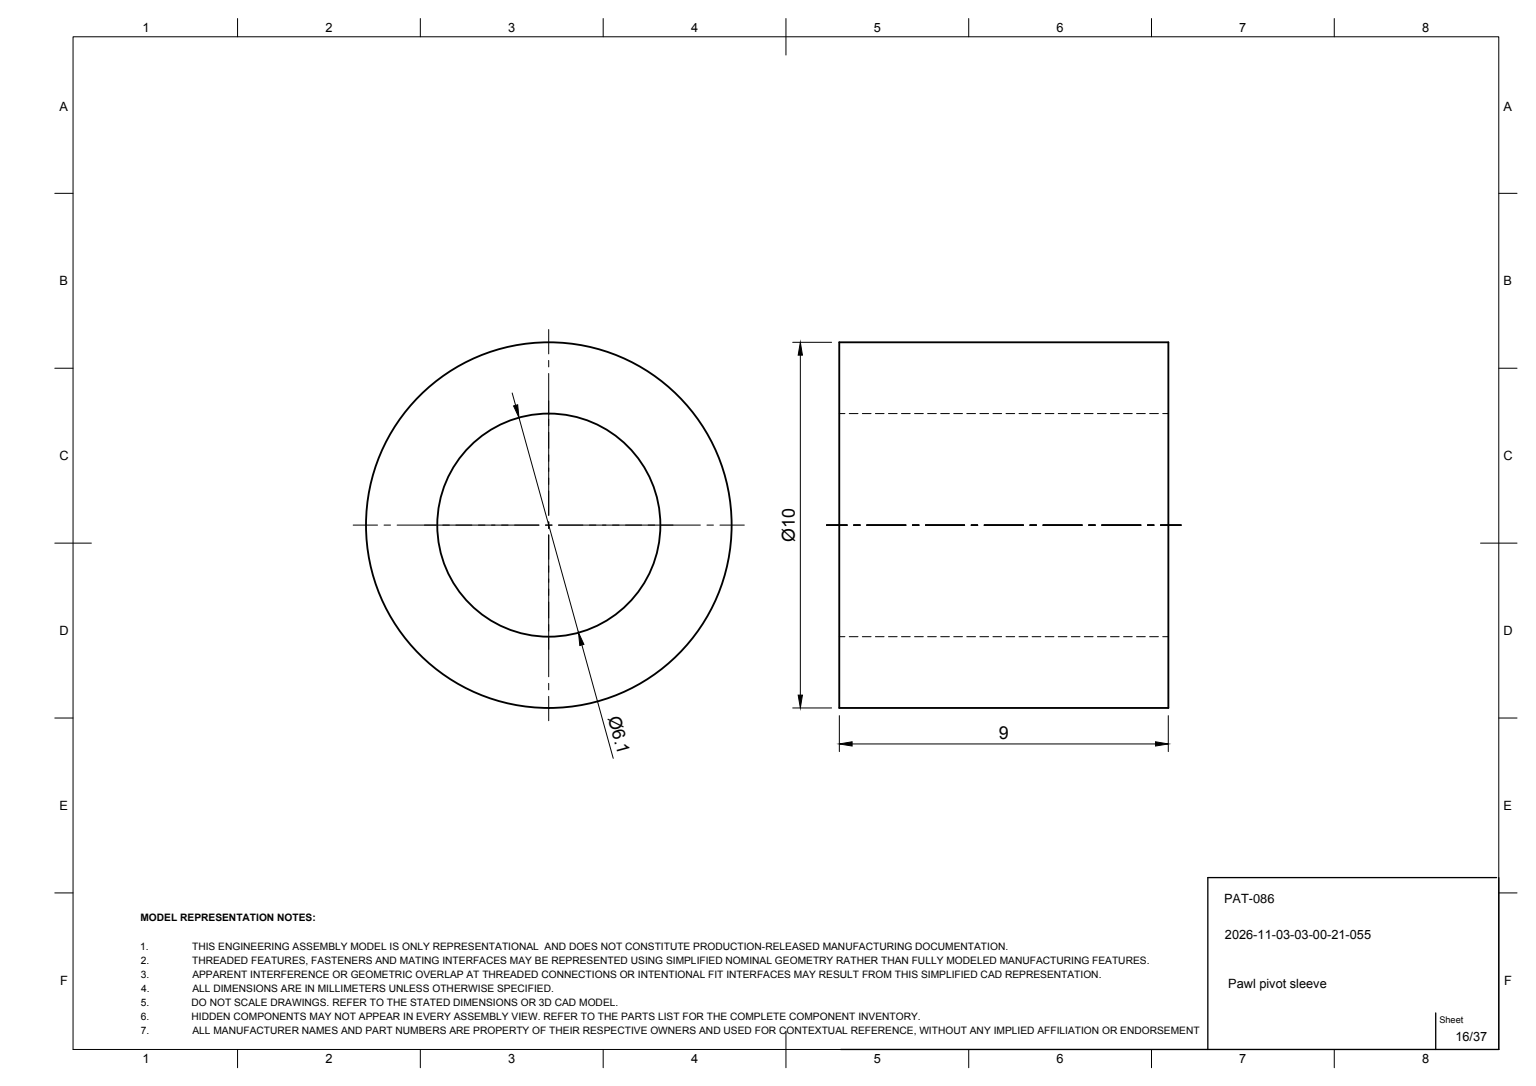
ISO-10303-21;
HEADER;
/* Generated by software containing ST-Developer
 * from STEP Tools, Inc. (www.steptools.com) 
 */

FILE_DESCRIPTION(
/* description */ ('Ratchet and pawl hand winch drum'),
/* implementation_level */ '2;1');

FILE_NAME(
/* name */ 'Pawl pivot sleeve.step',
/* time_stamp */ '2026-10-27T12:42:58-07:00',
/* author */ (''),
/* organization */ (''),
/* preprocessor_version */ 'ST-DEVELOPER v20.2',
/* originating_system */ 'Autodesk Translation Framework v15.17.0.0',
/* authorisation */ '');

FILE_SCHEMA (('AUTOMOTIVE_DESIGN { 1 0 10303 214 3 1 1 }'));
ENDSEC;

DATA;
#10=MECHANICAL_DESIGN_GEOMETRIC_PRESENTATION_REPRESENTATION('',(#400),#11801);
#332=SHAPE_REPRESENTATION_RELATIONSHIP('SRR','None',#11958,#366);
#366=ADVANCED_BREP_SHAPE_REPRESENTATION('',(#435),#11775);
#400=STYLED_ITEM('',(#12227),#435);
#435=MANIFOLD_SOLID_BREP('Body1',#6277);
#525=FACE_BOUND('',#1373,.T.);
#526=FACE_BOUND('',#1375,.T.);
#662=PLANE('',#6892);
#663=PLANE('',#6893);
#945=FACE_OUTER_BOUND('',#1370,.T.);
#946=FACE_OUTER_BOUND('',#1371,.T.);
#947=FACE_OUTER_BOUND('',#1372,.T.);
#948=FACE_OUTER_BOUND('',#1374,.T.);
#1370=EDGE_LOOP('',(#4679,#4680,#4681,#4682));
#1371=EDGE_LOOP('',(#4683,#4684,#4685,#4686));
#1372=EDGE_LOOP('',(#4687));
#1373=EDGE_LOOP('',(#4688));
#1374=EDGE_LOOP('',(#4689));
#1375=EDGE_LOOP('',(#4690));
#1825=LINE('',#9710,#2336);
#1826=LINE('',#9716,#2337);
#2336=VECTOR('',#7904,0.305);
#2337=VECTOR('',#7911,0.5);
#2807=CIRCLE('',#6887,0.305);
#2808=CIRCLE('',#6888,0.305);
#2809=CIRCLE('',#6890,0.5);
#2810=CIRCLE('',#6891,0.5);
#3086=VERTEX_POINT('',#9707);
#3087=VERTEX_POINT('',#9709);
#3088=VERTEX_POINT('',#9713);
#3089=VERTEX_POINT('',#9715);
#3683=EDGE_CURVE('',#3086,#3086,#2807,.T.);
#3684=EDGE_CURVE('',#3086,#3087,#1825,.T.);
#3685=EDGE_CURVE('',#3087,#3087,#2808,.T.);
#3686=EDGE_CURVE('',#3088,#3088,#2809,.T.);
#3687=EDGE_CURVE('',#3088,#3089,#1826,.T.);
#3688=EDGE_CURVE('',#3089,#3089,#2810,.T.);
#4679=ORIENTED_EDGE('',*,*,#3683,.F.);
#4680=ORIENTED_EDGE('',*,*,#3684,.T.);
#4681=ORIENTED_EDGE('',*,*,#3685,.T.);
#4682=ORIENTED_EDGE('',*,*,#3684,.F.);
#4683=ORIENTED_EDGE('',*,*,#3686,.F.);
#4684=ORIENTED_EDGE('',*,*,#3687,.T.);
#4685=ORIENTED_EDGE('',*,*,#3688,.T.);
#4686=ORIENTED_EDGE('',*,*,#3687,.F.);
#4687=ORIENTED_EDGE('',*,*,#3686,.T.);
#4688=ORIENTED_EDGE('',*,*,#3683,.T.);
#4689=ORIENTED_EDGE('',*,*,#3688,.F.);
#4690=ORIENTED_EDGE('',*,*,#3685,.F.);
#5851=CYLINDRICAL_SURFACE('',#6886,0.305);
#5852=CYLINDRICAL_SURFACE('',#6889,0.5);
#6015=ADVANCED_FACE('',(#945),#5851,.F.);
#6016=ADVANCED_FACE('',(#946),#5852,.T.);
#6017=ADVANCED_FACE('',(#947,#525),#662,.T.);
#6018=ADVANCED_FACE('',(#948,#526),#663,.F.);
#6277=CLOSED_SHELL('',(#6015,#6016,#6017,#6018));
#6885=AXIS2_PLACEMENT_3D('',#9705,#7898,#7899);
#6886=AXIS2_PLACEMENT_3D('',#9706,#7900,#7901);
#6887=AXIS2_PLACEMENT_3D('',#9708,#7902,#7903);
#6888=AXIS2_PLACEMENT_3D('',#9711,#7905,#7906);
#6889=AXIS2_PLACEMENT_3D('',#9712,#7907,#7908);
#6890=AXIS2_PLACEMENT_3D('',#9714,#7909,#7910);
#6891=AXIS2_PLACEMENT_3D('',#9717,#7912,#7913);
#6892=AXIS2_PLACEMENT_3D('',#9718,#7914,#7915);
#6893=AXIS2_PLACEMENT_3D('',#9719,#7916,#7917);
#7898=DIRECTION('axis',(0.,0.,1.));
#7899=DIRECTION('refdir',(1.,0.,0.));
#7900=DIRECTION('center_axis',(0.,1.,0.));
#7901=DIRECTION('ref_axis',(1.,0.,0.));
#7902=DIRECTION('center_axis',(0.,-1.,0.));
#7903=DIRECTION('ref_axis',(1.,0.,0.));
#7904=DIRECTION('',(0.,-1.,0.));
#7905=DIRECTION('center_axis',(0.,-1.,0.));
#7906=DIRECTION('ref_axis',(1.,0.,0.));
#7907=DIRECTION('center_axis',(0.,1.,0.));
#7908=DIRECTION('ref_axis',(1.,0.,0.));
#7909=DIRECTION('center_axis',(0.,1.,0.));
#7910=DIRECTION('ref_axis',(1.,0.,0.));
#7911=DIRECTION('',(0.,-1.,0.));
#7912=DIRECTION('center_axis',(0.,1.,0.));
#7913=DIRECTION('ref_axis',(1.,0.,0.));
#7914=DIRECTION('center_axis',(0.,1.,0.));
#7915=DIRECTION('ref_axis',(1.,0.,0.));
#7916=DIRECTION('center_axis',(0.,1.,0.));
#7917=DIRECTION('ref_axis',(1.,0.,0.));
#9705=CARTESIAN_POINT('',(0.,0.,0.));
#9706=CARTESIAN_POINT('Origin',(6.5,-4.4,10.));
#9707=CARTESIAN_POINT('',(6.195,-3.5,10.));
#9708=CARTESIAN_POINT('Origin',(6.5,-3.5,10.));
#9709=CARTESIAN_POINT('',(6.195,-4.4,10.));
#9710=CARTESIAN_POINT('',(6.195,-4.4,10.));
#9711=CARTESIAN_POINT('Origin',(6.5,-4.4,10.));
#9712=CARTESIAN_POINT('Origin',(6.5,-4.4,10.));
#9713=CARTESIAN_POINT('',(6.,-3.5,10.));
#9714=CARTESIAN_POINT('Origin',(6.5,-3.5,10.));
#9715=CARTESIAN_POINT('',(6.,-4.4,10.));
#9716=CARTESIAN_POINT('',(6.,-4.4,10.));
#9717=CARTESIAN_POINT('Origin',(6.5,-4.4,10.));
#9718=CARTESIAN_POINT('Origin',(6.5,-3.5,10.));
#9719=CARTESIAN_POINT('Origin',(6.5,-4.4,10.));
#11735=UNCERTAINTY_MEASURE_WITH_UNIT(LENGTH_MEASURE(0.001),#11802,
'DISTANCE_ACCURACY_VALUE',
'Maximum model space distance between geometric entities at asserted c
onnectivities');
#11761=UNCERTAINTY_MEASURE_WITH_UNIT(LENGTH_MEASURE(0.001),#11802,
'DISTANCE_ACCURACY_VALUE',
'Maximum model space distance between geometric entities at asserted c
onnectivities');
#11775=(
GEOMETRIC_REPRESENTATION_CONTEXT(3)
GLOBAL_UNCERTAINTY_ASSIGNED_CONTEXT((#11735))
GLOBAL_UNIT_ASSIGNED_CONTEXT((#11802,#11804,#11805))
REPRESENTATION_CONTEXT('','3D')
);
#11801=(
GEOMETRIC_REPRESENTATION_CONTEXT(3)
GLOBAL_UNCERTAINTY_ASSIGNED_CONTEXT((#11761))
GLOBAL_UNIT_ASSIGNED_CONTEXT((#11802,#11804,#11805))
REPRESENTATION_CONTEXT('','3D')
);
#11802=(
LENGTH_UNIT()
NAMED_UNIT(*)
SI_UNIT(.CENTI.,.METRE.)
);
#11804=(
NAMED_UNIT(*)
PLANE_ANGLE_UNIT()
SI_UNIT($,.RADIAN.)
);
#11805=(
NAMED_UNIT(*)
SI_UNIT($,.STERADIAN.)
SOLID_ANGLE_UNIT()
);
#11819=SHAPE_DEFINITION_REPRESENTATION(#11858,#11958);
#11858=PRODUCT_DEFINITION_SHAPE('',$,#11998);
#11958=SHAPE_REPRESENTATION('',(#6885),#11775);
#11984=PRODUCT_DEFINITION_CONTEXT('part definition',#12103,'design');
#11998=PRODUCT_DEFINITION('Pawl pivot sleeve','Pawl pivot sleeve',#12037,
#11984);
#12037=PRODUCT_DEFINITION_FORMATION('',$,#12118);
#12103=APPLICATION_CONTEXT(
'Core Data for Automotive Mechanical Design Process');
#12104=PRODUCT_CONTEXT('part definition',#12103,'mechanical');
#12118=PRODUCT('Pawl pivot sleeve','Pawl pivot sleeve',
'Pawl pivot sleeve',(#12104));
#12221=COLOUR_RGB('Off White',0.89,0.88,0.83);
#12222=FILL_AREA_STYLE_COLOUR('',#12221);
#12223=FILL_AREA_STYLE('',(#12222));
#12224=SURFACE_STYLE_FILL_AREA(#12223);
#12225=SURFACE_SIDE_STYLE('',(#12224));
#12226=SURFACE_STYLE_USAGE(.BOTH.,#12225);
#12227=PRESENTATION_STYLE_ASSIGNMENT((#12226));
ENDSEC;
END-ISO-10303-21;
